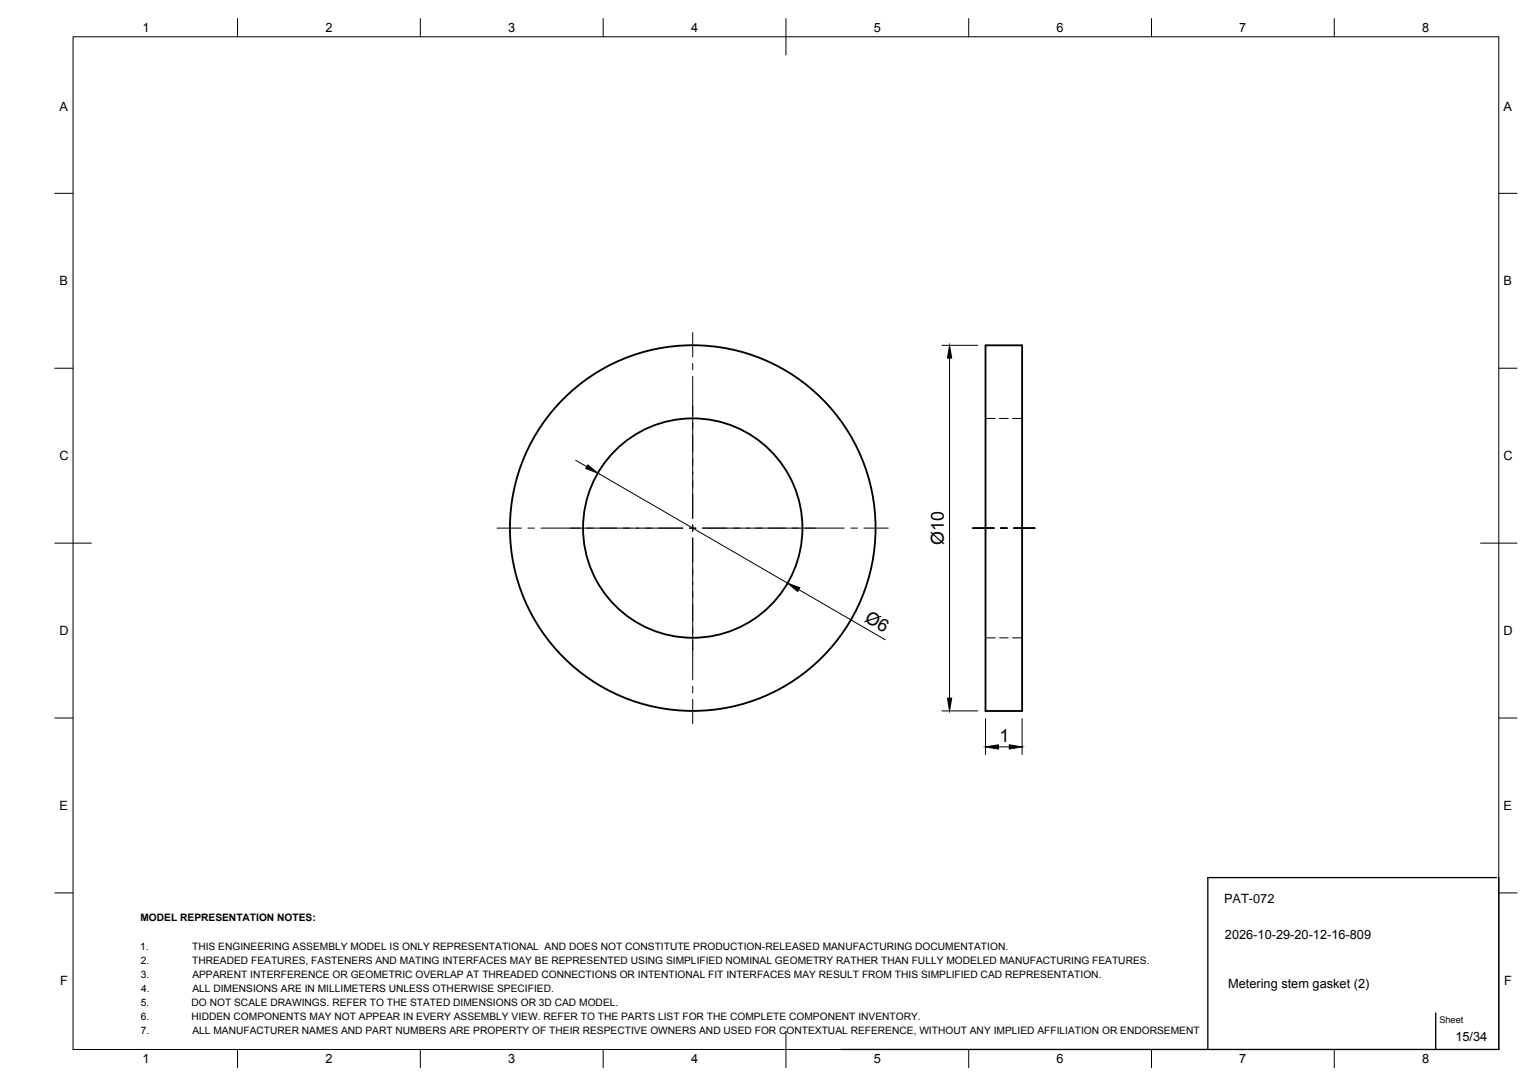
ISO-10303-21;
HEADER;
/* Generated by software containing ST-Developer
 * from STEP Tools, Inc. (www.steptools.com) 
 */

FILE_DESCRIPTION(
/* description */ ('PAT-072'),
/* implementation_level */ '2;1');

FILE_NAME(
/* name */ 'Metering stem gasket (2).step',
/* time_stamp */ '2026-10-29T20:11:56-07:00',
/* author */ (''),
/* organization */ (''),
/* preprocessor_version */ 'ST-DEVELOPER v20.2',
/* originating_system */ 'Autodesk Translation Framework v15.17.0.0',
/* authorisation */ '');

FILE_SCHEMA (('AUTOMOTIVE_DESIGN { 1 0 10303 214 3 1 1 }'));
ENDSEC;

DATA;
#10=MECHANICAL_DESIGN_GEOMETRIC_PRESENTATION_REPRESENTATION('',(#344),#11432);
#272=SHAPE_REPRESENTATION_RELATIONSHIP('SRR','None',#11576,#308);
#308=ADVANCED_BREP_SHAPE_REPRESENTATION('',(#380),#11407);
#344=STYLED_ITEM('',(#11833),#380);
#380=MANIFOLD_SOLID_BREP('Body1',#6079);
#476=FACE_BOUND('',#1383,.T.);
#477=FACE_BOUND('',#1385,.T.);
#643=PLANE('',#6786);
#644=PLANE('',#6787);
#934=FACE_OUTER_BOUND('',#1380,.T.);
#935=FACE_OUTER_BOUND('',#1381,.T.);
#936=FACE_OUTER_BOUND('',#1382,.T.);
#937=FACE_OUTER_BOUND('',#1384,.T.);
#1380=EDGE_LOOP('',(#4612,#4613,#4614,#4615));
#1381=EDGE_LOOP('',(#4616,#4617,#4618,#4619));
#1382=EDGE_LOOP('',(#4620));
#1383=EDGE_LOOP('',(#4621));
#1384=EDGE_LOOP('',(#4622));
#1385=EDGE_LOOP('',(#4623));
#1829=LINE('',#10137,#2248);
#1830=LINE('',#10143,#2249);
#2248=VECTOR('',#7940,0.3);
#2249=VECTOR('',#7947,0.5);
#2665=CIRCLE('',#6781,0.3);
#2666=CIRCLE('',#6782,0.3);
#2667=CIRCLE('',#6784,0.5);
#2668=CIRCLE('',#6785,0.5);
#3014=VERTEX_POINT('',#10134);
#3015=VERTEX_POINT('',#10136);
#3016=VERTEX_POINT('',#10140);
#3017=VERTEX_POINT('',#10142);
#3595=EDGE_CURVE('',#3014,#3014,#2665,.T.);
#3596=EDGE_CURVE('',#3014,#3015,#1829,.T.);
#3597=EDGE_CURVE('',#3015,#3015,#2666,.T.);
#3598=EDGE_CURVE('',#3016,#3016,#2667,.T.);
#3599=EDGE_CURVE('',#3016,#3017,#1830,.T.);
#3600=EDGE_CURVE('',#3017,#3017,#2668,.T.);
#4612=ORIENTED_EDGE('',*,*,#3595,.F.);
#4613=ORIENTED_EDGE('',*,*,#3596,.T.);
#4614=ORIENTED_EDGE('',*,*,#3597,.T.);
#4615=ORIENTED_EDGE('',*,*,#3596,.F.);
#4616=ORIENTED_EDGE('',*,*,#3598,.F.);
#4617=ORIENTED_EDGE('',*,*,#3599,.T.);
#4618=ORIENTED_EDGE('',*,*,#3600,.T.);
#4619=ORIENTED_EDGE('',*,*,#3599,.F.);
#4620=ORIENTED_EDGE('',*,*,#3598,.T.);
#4621=ORIENTED_EDGE('',*,*,#3595,.T.);
#4622=ORIENTED_EDGE('',*,*,#3600,.F.);
#4623=ORIENTED_EDGE('',*,*,#3597,.F.);
#5623=CYLINDRICAL_SURFACE('',#6780,0.3);
#5624=CYLINDRICAL_SURFACE('',#6783,0.5);
#5833=ADVANCED_FACE('',(#934),#5623,.F.);
#5834=ADVANCED_FACE('',(#935),#5624,.T.);
#5835=ADVANCED_FACE('',(#936,#476),#643,.T.);
#5836=ADVANCED_FACE('',(#937,#477),#644,.F.);
#6079=CLOSED_SHELL('',(#5833,#5834,#5835,#5836));
#6779=AXIS2_PLACEMENT_3D('',#10132,#7934,#7935);
#6780=AXIS2_PLACEMENT_3D('',#10133,#7936,#7937);
#6781=AXIS2_PLACEMENT_3D('',#10135,#7938,#7939);
#6782=AXIS2_PLACEMENT_3D('',#10138,#7941,#7942);
#6783=AXIS2_PLACEMENT_3D('',#10139,#7943,#7944);
#6784=AXIS2_PLACEMENT_3D('',#10141,#7945,#7946);
#6785=AXIS2_PLACEMENT_3D('',#10144,#7948,#7949);
#6786=AXIS2_PLACEMENT_3D('',#10145,#7950,#7951);
#6787=AXIS2_PLACEMENT_3D('',#10146,#7952,#7953);
#7934=DIRECTION('axis',(0.,0.,1.));
#7935=DIRECTION('refdir',(1.,0.,0.));
#7936=DIRECTION('center_axis',(0.,0.,1.));
#7937=DIRECTION('ref_axis',(1.,0.,0.));
#7938=DIRECTION('center_axis',(0.,0.,-1.));
#7939=DIRECTION('ref_axis',(1.,0.,0.));
#7940=DIRECTION('',(0.,0.,-1.));
#7941=DIRECTION('center_axis',(0.,0.,-1.));
#7942=DIRECTION('ref_axis',(1.,0.,0.));
#7943=DIRECTION('center_axis',(0.,0.,1.));
#7944=DIRECTION('ref_axis',(1.,0.,0.));
#7945=DIRECTION('center_axis',(0.,0.,1.));
#7946=DIRECTION('ref_axis',(1.,0.,0.));
#7947=DIRECTION('',(0.,0.,-1.));
#7948=DIRECTION('center_axis',(0.,0.,1.));
#7949=DIRECTION('ref_axis',(1.,0.,0.));
#7950=DIRECTION('center_axis',(0.,0.,1.));
#7951=DIRECTION('ref_axis',(1.,0.,0.));
#7952=DIRECTION('center_axis',(0.,0.,1.));
#7953=DIRECTION('ref_axis',(1.,0.,0.));
#10132=CARTESIAN_POINT('',(0.,0.,0.));
#10133=CARTESIAN_POINT('Origin',(1.25,1.5,6.));
#10134=CARTESIAN_POINT('',(0.95,1.5,6.1));
#10135=CARTESIAN_POINT('Origin',(1.25,1.5,6.1));
#10136=CARTESIAN_POINT('',(0.95,1.5,6.));
#10137=CARTESIAN_POINT('',(0.95,1.5,6.));
#10138=CARTESIAN_POINT('Origin',(1.25,1.5,6.));
#10139=CARTESIAN_POINT('Origin',(1.25,1.5,6.));
#10140=CARTESIAN_POINT('',(0.75,1.5,6.1));
#10141=CARTESIAN_POINT('Origin',(1.25,1.5,6.1));
#10142=CARTESIAN_POINT('',(0.75,1.5,6.));
#10143=CARTESIAN_POINT('',(0.75,1.5,6.));
#10144=CARTESIAN_POINT('Origin',(1.25,1.5,6.));
#10145=CARTESIAN_POINT('Origin',(1.25,1.5,6.1));
#10146=CARTESIAN_POINT('Origin',(1.25,1.5,6.));
#11368=UNCERTAINTY_MEASURE_WITH_UNIT(LENGTH_MEASURE(0.001),#11433,
'DISTANCE_ACCURACY_VALUE',
'Maximum model space distance between geometric entities at asserted c
onnectivities');
#11393=UNCERTAINTY_MEASURE_WITH_UNIT(LENGTH_MEASURE(0.001),#11433,
'DISTANCE_ACCURACY_VALUE',
'Maximum model space distance between geometric entities at asserted c
onnectivities');
#11407=(
GEOMETRIC_REPRESENTATION_CONTEXT(3)
GLOBAL_UNCERTAINTY_ASSIGNED_CONTEXT((#11368))
GLOBAL_UNIT_ASSIGNED_CONTEXT((#11433,#11435,#11436))
REPRESENTATION_CONTEXT('','3D')
);
#11432=(
GEOMETRIC_REPRESENTATION_CONTEXT(3)
GLOBAL_UNCERTAINTY_ASSIGNED_CONTEXT((#11393))
GLOBAL_UNIT_ASSIGNED_CONTEXT((#11433,#11435,#11436))
REPRESENTATION_CONTEXT('','3D')
);
#11433=(
LENGTH_UNIT()
NAMED_UNIT(*)
SI_UNIT(.CENTI.,.METRE.)
);
#11435=(
NAMED_UNIT(*)
PLANE_ANGLE_UNIT()
SI_UNIT($,.RADIAN.)
);
#11436=(
NAMED_UNIT(*)
SI_UNIT($,.STERADIAN.)
SOLID_ANGLE_UNIT()
);
#11450=SHAPE_DEFINITION_REPRESENTATION(#11488,#11576);
#11488=PRODUCT_DEFINITION_SHAPE('',$,#11615);
#11576=SHAPE_REPRESENTATION('',(#6779),#11407);
#11601=PRODUCT_DEFINITION_CONTEXT('part definition',#11717,'design');
#11615=PRODUCT_DEFINITION('Metering stem gasket (2)',
'Metering stem gasket (2)',#11653,#11601);
#11653=PRODUCT_DEFINITION_FORMATION('',$,#11732);
#11717=APPLICATION_CONTEXT(
'Core Data for Automotive Mechanical Design Process');
#11718=PRODUCT_CONTEXT('part definition',#11717,'mechanical');
#11732=PRODUCT('Metering stem gasket (2)','Metering stem gasket (2)',
'Metering stem gasket (2)',(#11718));
#11827=COLOUR_RGB('Off White',0.89,0.88,0.83);
#11828=FILL_AREA_STYLE_COLOUR('',#11827);
#11829=FILL_AREA_STYLE('',(#11828));
#11830=SURFACE_STYLE_FILL_AREA(#11829);
#11831=SURFACE_SIDE_STYLE('',(#11830));
#11832=SURFACE_STYLE_USAGE(.BOTH.,#11831);
#11833=PRESENTATION_STYLE_ASSIGNMENT((#11832));
ENDSEC;
END-ISO-10303-21;
